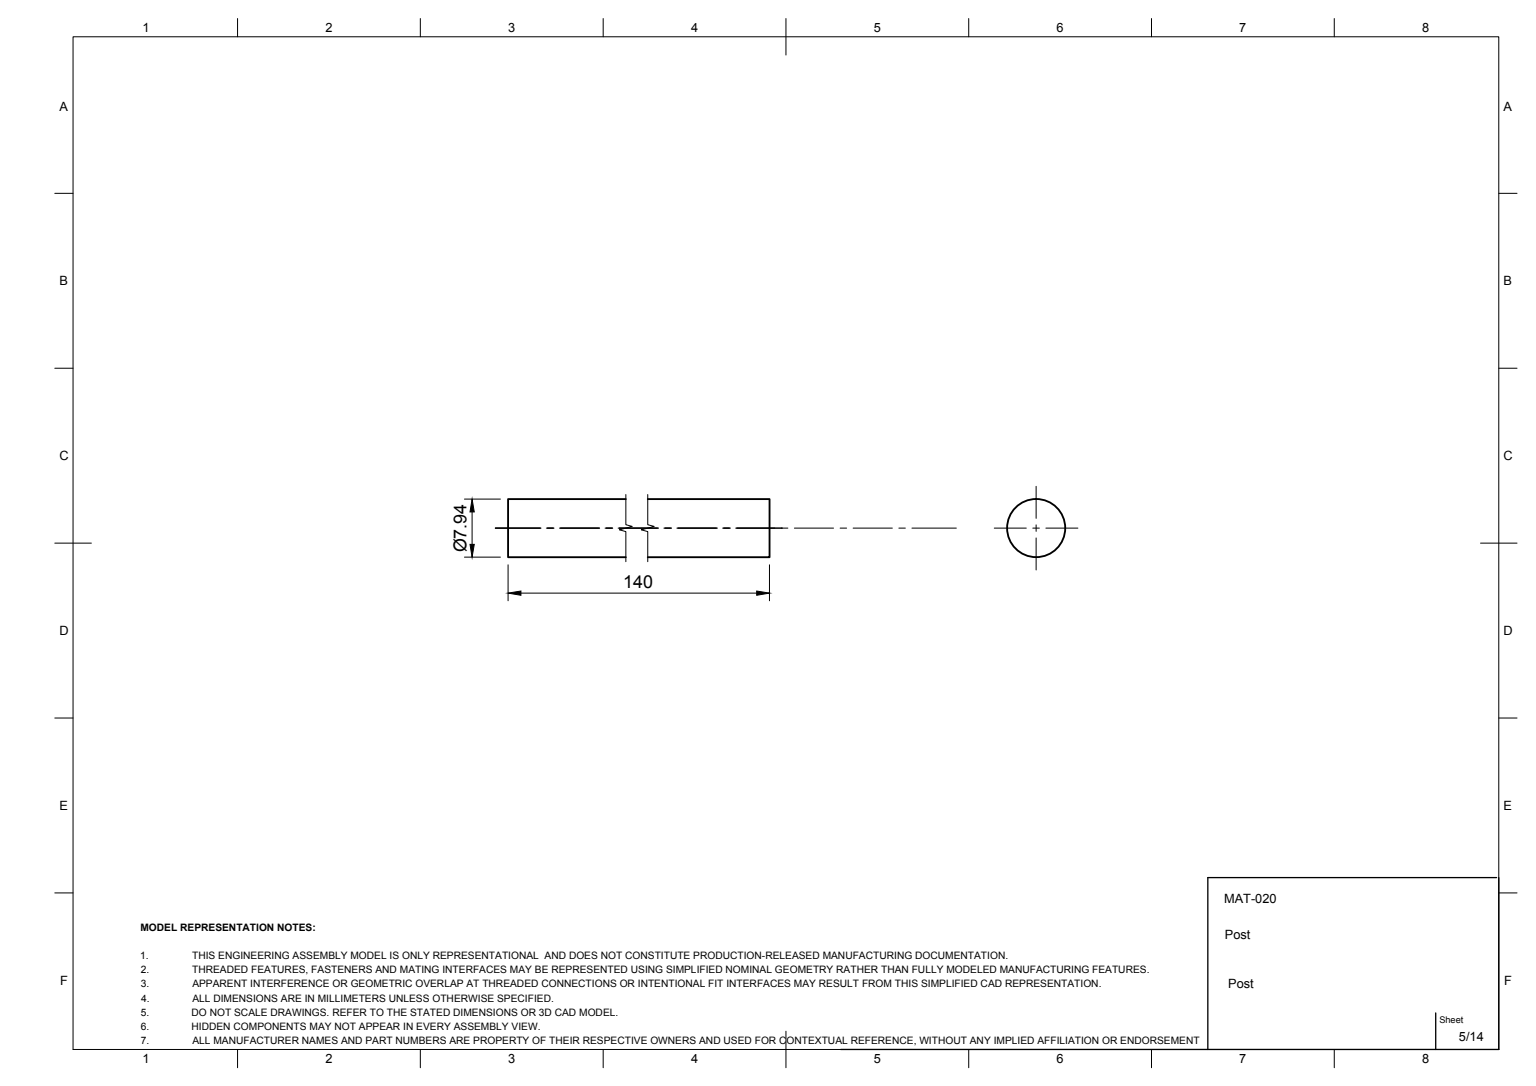
ISO-10303-21;
HEADER;
/* Generated by software containing ST-Developer
 * from STEP Tools, Inc. (www.steptools.com) 
 */

FILE_DESCRIPTION(
/* description */ ('STEP AP214'),
/* implementation_level */ '2;1');

FILE_NAME(
/* name */ 'Post.step',
/* time_stamp */ '2026-11-14T06:20:50-08:00',
/* author */ (''),
/* organization */ (''),
/* preprocessor_version */ 'ST-DEVELOPER v20.2',
/* originating_system */ 'Autodesk Translation Framework v15.17.0.0',
/* authorisation */ '');

FILE_SCHEMA (('AUTOMOTIVE_DESIGN { 1 0 10303 214 3 1 1 }'));
ENDSEC;

DATA;
#10=MECHANICAL_DESIGN_GEOMETRIC_PRESENTATION_REPRESENTATION('',(#966),#20658);
#437=PLANE('',#4070);
#438=PLANE('',#4071);
#628=LINE('',#20488,#821);
#821=VECTOR('',#4855,3.96875);
#929=CYLINDRICAL_SURFACE('',#4067,3.96875);
#942=SHAPE_REPRESENTATION_RELATIONSHIP('SRR','None',#20726,#954);
#954=ADVANCED_BREP_SHAPE_REPRESENTATION('',(#978),#20656);
#966=STYLED_ITEM('',(#20786),#978);
#978=MANIFOLD_SOLID_BREP('Body1',#3661);
#1173=FACE_OUTER_BOUND('',#1405,.T.);
#1174=FACE_OUTER_BOUND('',#1406,.T.);
#1175=FACE_OUTER_BOUND('',#1407,.T.);
#1405=EDGE_LOOP('',(#3368,#3369,#3370,#3371));
#1406=EDGE_LOOP('',(#3372));
#1407=EDGE_LOOP('',(#3373));
#1531=CIRCLE('',#4068,3.96875);
#1532=CIRCLE('',#4069,3.96875);
#1859=VERTEX_POINT('',#20485);
#1860=VERTEX_POINT('',#20487);
#2366=EDGE_CURVE('',#1859,#1859,#1531,.T.);
#2367=EDGE_CURVE('',#1859,#1860,#628,.T.);
#2368=EDGE_CURVE('',#1860,#1860,#1532,.T.);
#3368=ORIENTED_EDGE('',*,*,#2366,.T.);
#3369=ORIENTED_EDGE('',*,*,#2367,.T.);
#3370=ORIENTED_EDGE('',*,*,#2368,.F.);
#3371=ORIENTED_EDGE('',*,*,#2367,.F.);
#3372=ORIENTED_EDGE('',*,*,#2368,.T.);
#3373=ORIENTED_EDGE('',*,*,#2366,.F.);
#3635=ADVANCED_FACE('',(#1173),#929,.T.);
#3636=ADVANCED_FACE('',(#1174),#437,.T.);
#3637=ADVANCED_FACE('',(#1175),#438,.F.);
#3661=CLOSED_SHELL('',(#3635,#3636,#3637));
#4066=AXIS2_PLACEMENT_3D('',#20483,#4849,#4850);
#4067=AXIS2_PLACEMENT_3D('',#20484,#4851,#4852);
#4068=AXIS2_PLACEMENT_3D('',#20486,#4853,#4854);
#4069=AXIS2_PLACEMENT_3D('',#20489,#4856,#4857);
#4070=AXIS2_PLACEMENT_3D('',#20490,#4858,#4859);
#4071=AXIS2_PLACEMENT_3D('',#20491,#4860,#4861);
#4849=DIRECTION('axis',(0.,0.,1.));
#4850=DIRECTION('refdir',(1.,0.,0.));
#4851=DIRECTION('center_axis',(1.11022302462516E-16,-1.,0.));
#4852=DIRECTION('ref_axis',(0.,0.,-1.));
#4853=DIRECTION('center_axis',(-1.11022302462516E-16,1.,0.));
#4854=DIRECTION('ref_axis',(0.,0.,1.));
#4855=DIRECTION('',(-1.11022302462516E-16,1.,0.));
#4856=DIRECTION('center_axis',(-1.11022302462516E-16,1.,0.));
#4857=DIRECTION('ref_axis',(0.,0.,1.));
#4858=DIRECTION('center_axis',(-1.11022302462516E-16,1.,0.));
#4859=DIRECTION('ref_axis',(0.,0.,1.));
#4860=DIRECTION('center_axis',(-1.11022302462516E-16,1.,0.));
#4861=DIRECTION('ref_axis',(0.,0.,1.));
#20483=CARTESIAN_POINT('',(0.,0.,0.));
#20484=CARTESIAN_POINT('Origin',(6.93889390390723E-15,140.,0.));
#20485=CARTESIAN_POINT('',(2.19959845502478E-14,1.77635683940025E-14,3.96875));
#20486=CARTESIAN_POINT('Origin',(0.,0.,0.));
#20487=CARTESIAN_POINT('',(6.45286220549562E-15,140.,3.96875));
#20488=CARTESIAN_POINT('',(6.45286220549562E-15,140.,3.96875));
#20489=CARTESIAN_POINT('Origin',(6.93889390390723E-15,140.,0.));
#20490=CARTESIAN_POINT('Origin',(6.93889390390723E-15,140.,0.));
#20491=CARTESIAN_POINT('Origin',(0.,0.,0.));
#20642=UNCERTAINTY_MEASURE_WITH_UNIT(LENGTH_MEASURE(0.01),#20659,
'DISTANCE_ACCURACY_VALUE',
'Maximum model space distance between geometric entities at asserted c
onnectivities');
#20644=UNCERTAINTY_MEASURE_WITH_UNIT(LENGTH_MEASURE(0.01),#20659,
'DISTANCE_ACCURACY_VALUE',
'Maximum model space distance between geometric entities at asserted c
onnectivities');
#20656=(
GEOMETRIC_REPRESENTATION_CONTEXT(3)
GLOBAL_UNCERTAINTY_ASSIGNED_CONTEXT((#20642))
GLOBAL_UNIT_ASSIGNED_CONTEXT((#20659,#20661,#20662))
REPRESENTATION_CONTEXT('','3D')
);
#20658=(
GEOMETRIC_REPRESENTATION_CONTEXT(3)
GLOBAL_UNCERTAINTY_ASSIGNED_CONTEXT((#20644))
GLOBAL_UNIT_ASSIGNED_CONTEXT((#20659,#20661,#20662))
REPRESENTATION_CONTEXT('','3D')
);
#20659=(
LENGTH_UNIT()
NAMED_UNIT(*)
SI_UNIT(.MILLI.,.METRE.)
);
#20661=(
NAMED_UNIT(*)
PLANE_ANGLE_UNIT()
SI_UNIT($,.RADIAN.)
);
#20662=(
NAMED_UNIT(*)
SI_UNIT($,.STERADIAN.)
SOLID_ANGLE_UNIT()
);
#20674=SHAPE_DEFINITION_REPRESENTATION(#20687,#20726);
#20687=PRODUCT_DEFINITION_SHAPE('',$,#20740);
#20726=SHAPE_REPRESENTATION('',(#4066),#20656);
#20728=PRODUCT_DEFINITION_CONTEXT('part definition',#20769,'design');
#20740=PRODUCT_DEFINITION('Post','Post',#20753,#20728);
#20753=PRODUCT_DEFINITION_FORMATION('',$,#20782);
#20769=APPLICATION_CONTEXT(
'Core Data for Automotive Mechanical Design Process');
#20770=PRODUCT_CONTEXT('part definition',#20769,'mechanical');
#20782=PRODUCT('Post','Post',$,(#20770));
#20786=PRESENTATION_STYLE_ASSIGNMENT((#20791));
#20791=SURFACE_STYLE_USAGE(.BOTH.,#20796);
#20796=SURFACE_SIDE_STYLE('',(#20801));
#20801=SURFACE_STYLE_FILL_AREA(#20806);
#20806=FILL_AREA_STYLE('Opaque(61,176,222)',(#20811));
#20811=FILL_AREA_STYLE_COLOUR('Opaque(61,176,222)',#20816);
#20816=COLOUR_RGB('Opaque(61,176,222)',0.23921568627451,0.690196078431373,
0.870588235294118);
ENDSEC;
END-ISO-10303-21;
